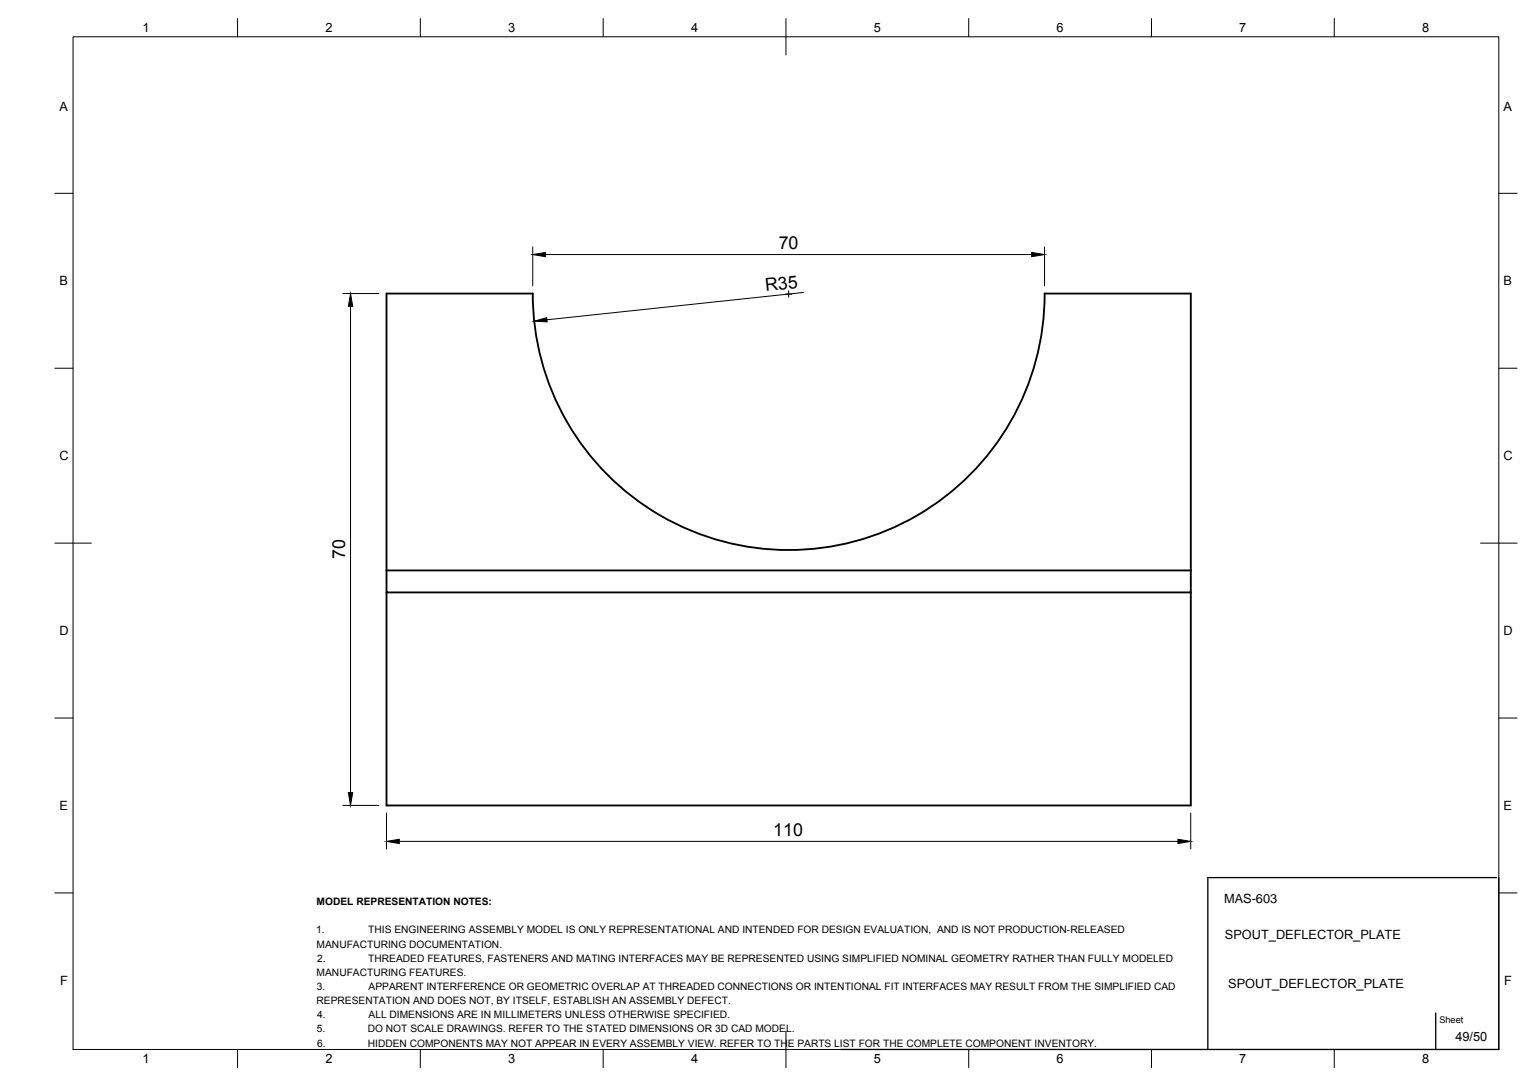
ISO-10303-21;
HEADER;
FILE_DESCRIPTION((''),'2;1');
FILE_NAME('SPOUT_DEFLECTOR_PLATE.step','2026-10-01T22:06:14-07:00',(''),(''),'','','');
FILE_SCHEMA (('AUTOMOTIVE_DESIGN { 1 0 10303 214 3 1 1 }'));
ENDSEC;
DATA;
#10=MECHANICAL_DESIGN_GEOMETRIC_PRESENTATION_REPRESENTATION('',(#1027,#1028),#50440);
#927=SHAPE_REPRESENTATION_RELATIONSHIP('SRR','None',#50661,#972) ;
#972=ADVANCED_BREP_SHAPE_REPRESENTATION('',(#1080,#1081),#50430) ;
#1027=STYLED_ITEM('',(#50889),#1080) ;
#1028=STYLED_ITEM('',(#50889),#1081) ;
#1080=MANIFOLD_SOLID_BREP('SPOUT_DEFLECTOR_PLATE',#28705) ;
#1081=MANIFOLD_SOLID_BREP('SPOUT_DEFLECTOR_PLATE',#28706) ;
#2276=PLANE('',#32170) ;
#2277=PLANE('',#32171) ;
#2278=PLANE('',#32172) ;
#2279=PLANE('',#32173) ;
#2280=PLANE('',#32174) ;
#2281=PLANE('',#32175) ;
#2282=PLANE('',#32176) ;
#2283=PLANE('',#32177) ;
#2284=PLANE('',#32178) ;
#2285=PLANE('',#32179) ;
#2286=PLANE('',#32180) ;
#2287=PLANE('',#32181) ;
#2288=PLANE('',#32182) ;
#3795=FACE_OUTER_BOUND('',#5635,.T.) ;
#3796=FACE_OUTER_BOUND('',#5636,.T.) ;
#3797=FACE_OUTER_BOUND('',#5637,.T.) ;
#3798=FACE_OUTER_BOUND('',#5638,.T.) ;
#3799=FACE_OUTER_BOUND('',#5639,.T.) ;
#3800=FACE_OUTER_BOUND('',#5640,.T.) ;
#3801=FACE_OUTER_BOUND('',#5641,.T.) ;
#3802=FACE_OUTER_BOUND('',#5642,.T.) ;
#3803=FACE_OUTER_BOUND('',#5643,.T.) ;
#3804=FACE_OUTER_BOUND('',#5644,.T.) ;
#3805=FACE_OUTER_BOUND('',#5645,.T.) ;
#3806=FACE_OUTER_BOUND('',#5646,.T.) ;
#3807=FACE_OUTER_BOUND('',#5647,.T.) ;
#3808=FACE_OUTER_BOUND('',#5648,.T.) ;
#5635=EDGE_LOOP('',(#26199,#26200,#26201,#26202)) ;
#5636=EDGE_LOOP('',(#26203,#26204,#26205,#26206,#26207,#26208)) ;
#5637=EDGE_LOOP('',(#26209,#26210,#26211,#26212)) ;
#5638=EDGE_LOOP('',(#26213,#26214,#26215,#26216)) ;
#5639=EDGE_LOOP('',(#26217,#26218,#26219,#26220)) ;
#5640=EDGE_LOOP('',(#26221,#26222,#26223,#26224)) ;
#5641=EDGE_LOOP('',(#26225,#26226,#26227,#26228)) ;
#5642=EDGE_LOOP('',(#26229,#26230,#26231,#26232,#26233,#26234)) ;
#5643=EDGE_LOOP('',(#26235,#26236,#26237,#26238)) ;
#5644=EDGE_LOOP('',(#26239,#26240,#26241,#26242)) ;
#5645=EDGE_LOOP('',(#26243,#26244,#26245,#26246)) ;
#5646=EDGE_LOOP('',(#26247,#26248,#26249,#26250)) ;
#5647=EDGE_LOOP('',(#26251,#26252,#26253,#26254)) ;
#5648=EDGE_LOOP('',(#26255,#26256,#26257,#26258)) ;
#8077=LINE('',#49780,#10549) ;
#8078=LINE('',#49784,#10550) ;
#8079=LINE('',#49788,#10551) ;
#8080=LINE('',#49790,#10552) ;
#8081=LINE('',#49792,#10553) ;
#8082=LINE('',#49794,#10554) ;
#8083=LINE('',#49795,#10555) ;
#8084=LINE('',#49798,#10556) ;
#8085=LINE('',#49799,#10557) ;
#8086=LINE('',#49802,#10558) ;
#8087=LINE('',#49803,#10559) ;
#8088=LINE('',#49807,#10560) ;
#8089=LINE('',#49808,#10561) ;
#8090=LINE('',#49809,#10562) ;
#8091=LINE('',#49811,#10563) ;
#8092=LINE('',#49813,#10564) ;
#8093=LINE('',#49818,#10565) ;
#8094=LINE('',#49820,#10566) ;
#8095=LINE('',#49822,#10567) ;
#8096=LINE('',#49823,#10568) ;
#8097=LINE('',#49827,#10569) ;
#8098=LINE('',#49829,#10570) ;
#8099=LINE('',#49831,#10571) ;
#8100=LINE('',#49832,#10572) ;
#8101=LINE('',#49834,#10573) ;
#8102=LINE('',#49835,#10574) ;
#8103=LINE('',#49837,#10575) ;
#8104=LINE('',#49839,#10576) ;
#10549=VECTOR('',#40638,1.) ;
#10550=VECTOR('',#40641,1.) ;
#10551=VECTOR('',#40646,1.) ;
#10552=VECTOR('',#40647,1.) ;
#10553=VECTOR('',#40648,1.) ;
#10554=VECTOR('',#40649,1.) ;
#10555=VECTOR('',#40650,1.) ;
#10556=VECTOR('',#40653,1.) ;
#10557=VECTOR('',#40654,1.) ;
#10558=VECTOR('',#40657,1.) ;
#10559=VECTOR('',#40658,1.) ;
#10560=VECTOR('',#40661,1.) ;
#10561=VECTOR('',#40662,1.) ;
#10562=VECTOR('',#40663,1.) ;
#10563=VECTOR('',#40666,1.) ;
#10564=VECTOR('',#40669,1.) ;
#10565=VECTOR('',#40674,1.) ;
#10566=VECTOR('',#40675,1.) ;
#10567=VECTOR('',#40676,1.) ;
#10568=VECTOR('',#40677,1.) ;
#10569=VECTOR('',#40680,1.) ;
#10570=VECTOR('',#40681,1.) ;
#10571=VECTOR('',#40682,1.) ;
#10572=VECTOR('',#40683,1.) ;
#10573=VECTOR('',#40686,1.) ;
#10574=VECTOR('',#40687,1.) ;
#10575=VECTOR('',#40690,1.) ;
#10576=VECTOR('',#40693,1.) ;
#11795=CIRCLE('',#32168,3.5) ;
#11796=CIRCLE('',#32169,3.5) ;
#14412=VERTEX_POINT('',#49778) ;
#14413=VERTEX_POINT('',#49779) ;
#14414=VERTEX_POINT('',#49781) ;
#14415=VERTEX_POINT('',#49783) ;
#14416=VERTEX_POINT('',#49787) ;
#14417=VERTEX_POINT('',#49789) ;
#14418=VERTEX_POINT('',#49791) ;
#14419=VERTEX_POINT('',#49793) ;
#14420=VERTEX_POINT('',#49797) ;
#14421=VERTEX_POINT('',#49801) ;
#14422=VERTEX_POINT('',#49805) ;
#14423=VERTEX_POINT('',#49806) ;
#14424=VERTEX_POINT('',#49816) ;
#14425=VERTEX_POINT('',#49817) ;
#14426=VERTEX_POINT('',#49819) ;
#14427=VERTEX_POINT('',#49821) ;
#14428=VERTEX_POINT('',#49825) ;
#14429=VERTEX_POINT('',#49826) ;
#14430=VERTEX_POINT('',#49828) ;
#14431=VERTEX_POINT('',#49830) ;
#18365=EDGE_CURVE('',#14412,#14413,#8077,.T.) ;
#18366=EDGE_CURVE('',#14414,#14412,#11795,.T.) ;
#18367=EDGE_CURVE('',#14415,#14414,#8078,.T.) ;
#18368=EDGE_CURVE('',#14413,#14415,#11796,.T.) ;
#18369=EDGE_CURVE('',#14416,#14412,#8079,.T.) ;
#18370=EDGE_CURVE('',#14416,#14417,#8080,.T.) ;
#18371=EDGE_CURVE('',#14418,#14417,#8081,.T.) ;
#18372=EDGE_CURVE('',#14419,#14418,#8082,.T.) ;
#18373=EDGE_CURVE('',#14414,#14419,#8083,.T.) ;
#18374=EDGE_CURVE('',#14413,#14420,#8084,.T.) ;
#18375=EDGE_CURVE('',#14420,#14416,#8085,.T.) ;
#18376=EDGE_CURVE('',#14419,#14421,#8086,.T.) ;
#18377=EDGE_CURVE('',#14421,#14415,#8087,.T.) ;
#18378=EDGE_CURVE('',#14422,#14423,#8088,.T.) ;
#18379=EDGE_CURVE('',#14423,#14418,#8089,.T.) ;
#18380=EDGE_CURVE('',#14417,#14422,#8090,.T.) ;
#18381=EDGE_CURVE('',#14421,#14423,#8091,.T.) ;
#18382=EDGE_CURVE('',#14420,#14422,#8092,.T.) ;
#18383=EDGE_CURVE('',#14424,#14425,#8093,.T.) ;
#18384=EDGE_CURVE('',#14425,#14426,#8094,.T.) ;
#18385=EDGE_CURVE('',#14426,#14427,#8095,.T.) ;
#18386=EDGE_CURVE('',#14427,#14424,#8096,.T.) ;
#18387=EDGE_CURVE('',#14428,#14429,#8097,.T.) ;
#18388=EDGE_CURVE('',#14429,#14430,#8098,.T.) ;
#18389=EDGE_CURVE('',#14430,#14431,#8099,.T.) ;
#18390=EDGE_CURVE('',#14431,#14428,#8100,.T.) ;
#18391=EDGE_CURVE('',#14427,#14430,#8101,.T.) ;
#18392=EDGE_CURVE('',#14424,#14429,#8102,.T.) ;
#18393=EDGE_CURVE('',#14426,#14431,#8103,.T.) ;
#18394=EDGE_CURVE('',#14425,#14428,#8104,.T.) ;
#26199=ORIENTED_EDGE('',*,*,#18365,.F.) ;
#26200=ORIENTED_EDGE('',*,*,#18366,.F.) ;
#26201=ORIENTED_EDGE('',*,*,#18367,.F.) ;
#26202=ORIENTED_EDGE('',*,*,#18368,.F.) ;
#26203=ORIENTED_EDGE('',*,*,#18366,.T.) ;
#26204=ORIENTED_EDGE('',*,*,#18369,.F.) ;
#26205=ORIENTED_EDGE('',*,*,#18370,.T.) ;
#26206=ORIENTED_EDGE('',*,*,#18371,.F.) ;
#26207=ORIENTED_EDGE('',*,*,#18372,.F.) ;
#26208=ORIENTED_EDGE('',*,*,#18373,.F.) ;
#26209=ORIENTED_EDGE('',*,*,#18365,.T.) ;
#26210=ORIENTED_EDGE('',*,*,#18374,.T.) ;
#26211=ORIENTED_EDGE('',*,*,#18375,.T.) ;
#26212=ORIENTED_EDGE('',*,*,#18369,.T.) ;
#26213=ORIENTED_EDGE('',*,*,#18367,.T.) ;
#26214=ORIENTED_EDGE('',*,*,#18373,.T.) ;
#26215=ORIENTED_EDGE('',*,*,#18376,.T.) ;
#26216=ORIENTED_EDGE('',*,*,#18377,.T.) ;
#26217=ORIENTED_EDGE('',*,*,#18378,.T.) ;
#26218=ORIENTED_EDGE('',*,*,#18379,.T.) ;
#26219=ORIENTED_EDGE('',*,*,#18371,.T.) ;
#26220=ORIENTED_EDGE('',*,*,#18380,.T.) ;
#26221=ORIENTED_EDGE('',*,*,#18372,.T.) ;
#26222=ORIENTED_EDGE('',*,*,#18379,.F.) ;
#26223=ORIENTED_EDGE('',*,*,#18381,.F.) ;
#26224=ORIENTED_EDGE('',*,*,#18376,.F.) ;
#26225=ORIENTED_EDGE('',*,*,#18382,.T.) ;
#26226=ORIENTED_EDGE('',*,*,#18380,.F.) ;
#26227=ORIENTED_EDGE('',*,*,#18370,.F.) ;
#26228=ORIENTED_EDGE('',*,*,#18375,.F.) ;
#26229=ORIENTED_EDGE('',*,*,#18368,.T.) ;
#26230=ORIENTED_EDGE('',*,*,#18377,.F.) ;
#26231=ORIENTED_EDGE('',*,*,#18381,.T.) ;
#26232=ORIENTED_EDGE('',*,*,#18378,.F.) ;
#26233=ORIENTED_EDGE('',*,*,#18382,.F.) ;
#26234=ORIENTED_EDGE('',*,*,#18374,.F.) ;
#26235=ORIENTED_EDGE('',*,*,#18383,.T.) ;
#26236=ORIENTED_EDGE('',*,*,#18384,.T.) ;
#26237=ORIENTED_EDGE('',*,*,#18385,.T.) ;
#26238=ORIENTED_EDGE('',*,*,#18386,.T.) ;
#26239=ORIENTED_EDGE('',*,*,#18387,.T.) ;
#26240=ORIENTED_EDGE('',*,*,#18388,.T.) ;
#26241=ORIENTED_EDGE('',*,*,#18389,.T.) ;
#26242=ORIENTED_EDGE('',*,*,#18390,.T.) ;
#26243=ORIENTED_EDGE('',*,*,#18391,.T.) ;
#26244=ORIENTED_EDGE('',*,*,#18388,.F.) ;
#26245=ORIENTED_EDGE('',*,*,#18392,.F.) ;
#26246=ORIENTED_EDGE('',*,*,#18386,.F.) ;
#26247=ORIENTED_EDGE('',*,*,#18393,.T.) ;
#26248=ORIENTED_EDGE('',*,*,#18389,.F.) ;
#26249=ORIENTED_EDGE('',*,*,#18391,.F.) ;
#26250=ORIENTED_EDGE('',*,*,#18385,.F.) ;
#26251=ORIENTED_EDGE('',*,*,#18394,.T.) ;
#26252=ORIENTED_EDGE('',*,*,#18390,.F.) ;
#26253=ORIENTED_EDGE('',*,*,#18393,.F.) ;
#26254=ORIENTED_EDGE('',*,*,#18384,.F.) ;
#26255=ORIENTED_EDGE('',*,*,#18392,.T.) ;
#26256=ORIENTED_EDGE('',*,*,#18387,.F.) ;
#26257=ORIENTED_EDGE('',*,*,#18394,.F.) ;
#26258=ORIENTED_EDGE('',*,*,#18383,.F.) ;
#27051=CYLINDRICAL_SURFACE('',#32167,3.5) ;
#28530=ADVANCED_FACE('',(#3795),#27051,.F.) ;
#28531=ADVANCED_FACE('',(#3796),#2276,.F.) ;
#28532=ADVANCED_FACE('',(#3797),#2277,.T.) ;
#28533=ADVANCED_FACE('',(#3798),#2278,.T.) ;
#28534=ADVANCED_FACE('',(#3799),#2279,.F.) ;
#28535=ADVANCED_FACE('',(#3800),#2280,.F.) ;
#28536=ADVANCED_FACE('',(#3801),#2281,.F.) ;
#28537=ADVANCED_FACE('',(#3802),#2282,.F.) ;
#28538=ADVANCED_FACE('',(#3803),#2283,.T.) ;
#28539=ADVANCED_FACE('',(#3804),#2284,.F.) ;
#28540=ADVANCED_FACE('',(#3805),#2285,.F.) ;
#28541=ADVANCED_FACE('',(#3806),#2286,.F.) ;
#28542=ADVANCED_FACE('',(#3807),#2287,.F.) ;
#28543=ADVANCED_FACE('',(#3808),#2288,.F.) ;
#28705=CLOSED_SHELL('',(#28530,#28531,#28532,#28533,#28534,#28535,#28536,
#28537)) ;
#28706=CLOSED_SHELL('',(#28538,#28539,#28540,#28541,#28542,#28543)) ;
#32166=AXIS2_PLACEMENT_3D('',#49776,#40634,#40635) ;
#32167=AXIS2_PLACEMENT_3D('',#49777,#40636,#40637) ;
#32168=AXIS2_PLACEMENT_3D('',#49782,#40639,#40640) ;
#32169=AXIS2_PLACEMENT_3D('',#49785,#40642,#40643) ;
#32170=AXIS2_PLACEMENT_3D('',#49786,#40644,#40645) ;
#32171=AXIS2_PLACEMENT_3D('',#49796,#40651,#40652) ;
#32172=AXIS2_PLACEMENT_3D('',#49800,#40655,#40656) ;
#32173=AXIS2_PLACEMENT_3D('',#49804,#40659,#40660) ;
#32174=AXIS2_PLACEMENT_3D('',#49810,#40664,#40665) ;
#32175=AXIS2_PLACEMENT_3D('',#49812,#40667,#40668) ;
#32176=AXIS2_PLACEMENT_3D('',#49814,#40670,#40671) ;
#32177=AXIS2_PLACEMENT_3D('',#49815,#40672,#40673) ;
#32178=AXIS2_PLACEMENT_3D('',#49824,#40678,#40679) ;
#32179=AXIS2_PLACEMENT_3D('',#49833,#40684,#40685) ;
#32180=AXIS2_PLACEMENT_3D('',#49836,#40688,#40689) ;
#32181=AXIS2_PLACEMENT_3D('',#49838,#40691,#40692) ;
#32182=AXIS2_PLACEMENT_3D('',#49840,#40694,#40695) ;
#40634=DIRECTION('axis',(0.,0.,1.)) ;
#40635=DIRECTION('refdir',(1.,0.,0.)) ;
#40636=DIRECTION('center_axis',(0.998052578482889,0.,-0.0623782861551805)) ;
#40637=DIRECTION('ref_axis',(-0.0623782861551805,1.22464679914735E-16,-0.998052578482889)) ;
#40638=DIRECTION('',(0.998052578482889,0.,-0.0623782861551805)) ;
#40639=DIRECTION('center_axis',(0.998052578482889,0.,-0.0623782861551805)) ;
#40640=DIRECTION('ref_axis',(0.0623782861551805,0.,0.998052578482889)) ;
#40641=DIRECTION('',(-0.998052578482889,0.,0.0623782861551805)) ;
#40642=DIRECTION('center_axis',(-0.998052578482889,0.,0.0623782861551805)) ;
#40643=DIRECTION('ref_axis',(0.0623782861551805,0.,0.998052578482889)) ;
#40644=DIRECTION('center_axis',(0.998052578482889,0.,-0.0623782861551805)) ;
#40645=DIRECTION('ref_axis',(-0.0623782861551805,0.,-0.998052578482889)) ;
#40646=DIRECTION('',(0.,-1.,0.)) ;
#40647=DIRECTION('',(-0.0623782861551805,0.,-0.998052578482889)) ;
#40648=DIRECTION('',(0.,1.,0.)) ;
#40649=DIRECTION('',(-0.0623782861551805,0.,-0.998052578482889)) ;
#40650=DIRECTION('',(0.,-1.,0.)) ;
#40651=DIRECTION('center_axis',(0.0623782861551805,0.,0.998052578482889)) ;
#40652=DIRECTION('ref_axis',(0.998052578482889,0.,-0.0623782861551805)) ;
#40653=DIRECTION('',(0.,1.,0.)) ;
#40654=DIRECTION('',(-0.998052578482889,0.,0.0623782861551805)) ;
#40655=DIRECTION('center_axis',(0.0623782861551805,0.,0.998052578482889)) ;
#40656=DIRECTION('ref_axis',(0.998052578482889,0.,-0.0623782861551805)) ;
#40657=DIRECTION('',(0.998052578482889,0.,-0.0623782861551805)) ;
#40658=DIRECTION('',(0.,1.,0.)) ;
#40659=DIRECTION('center_axis',(0.0623782861551805,0.,0.998052578482889)) ;
#40660=DIRECTION('ref_axis',(0.998052578482889,0.,-0.0623782861551805)) ;
#40661=DIRECTION('',(0.,-1.,0.)) ;
#40662=DIRECTION('',(-0.998052578482889,0.,0.0623782861551805)) ;
#40663=DIRECTION('',(0.998052578482889,0.,-0.0623782861551805)) ;
#40664=DIRECTION('center_axis',(0.,1.,0.)) ;
#40665=DIRECTION('ref_axis',(0.0623782861551805,0.,0.998052578482889)) ;
#40666=DIRECTION('',(-0.0623782861551805,0.,-0.998052578482889)) ;
#40667=DIRECTION('center_axis',(0.,-1.,0.)) ;
#40668=DIRECTION('ref_axis',(-0.0623782861551805,0.,-0.998052578482889)) ;
#40669=DIRECTION('',(-0.0623782861551805,0.,-0.998052578482889)) ;
#40670=DIRECTION('center_axis',(-0.998052578482889,0.,0.0623782861551805)) ;
#40671=DIRECTION('ref_axis',(0.0623782861551805,0.,0.998052578482889)) ;
#40672=DIRECTION('center_axis',(0.0623782861551805,0.,0.998052578482889)) ;
#40673=DIRECTION('ref_axis',(0.998052578482889,0.,-0.0623782861551805)) ;
#40674=DIRECTION('',(0.,1.,0.)) ;
#40675=DIRECTION('',(-0.998052578482889,0.,0.0623782861551805)) ;
#40676=DIRECTION('',(0.,-1.,0.)) ;
#40677=DIRECTION('',(0.998052578482889,0.,-0.0623782861551805)) ;
#40678=DIRECTION('center_axis',(0.0623782861551805,0.,0.998052578482889)) ;
#40679=DIRECTION('ref_axis',(0.998052578482889,0.,-0.0623782861551805)) ;
#40680=DIRECTION('',(0.,-1.,0.)) ;
#40681=DIRECTION('',(-0.998052578482889,0.,0.0623782861551805)) ;
#40682=DIRECTION('',(0.,1.,0.)) ;
#40683=DIRECTION('',(0.998052578482889,0.,-0.0623782861551805)) ;
#40684=DIRECTION('center_axis',(0.,1.,0.)) ;
#40685=DIRECTION('ref_axis',(0.0623782861551805,0.,0.998052578482889)) ;
#40686=DIRECTION('',(-0.0623782861551805,0.,-0.998052578482889)) ;
#40687=DIRECTION('',(-0.0623782861551805,0.,-0.998052578482889)) ;
#40688=DIRECTION('center_axis',(0.998052578482889,0.,-0.0623782861551805)) ;
#40689=DIRECTION('ref_axis',(-0.0623782861551805,0.,-0.998052578482889)) ;
#40690=DIRECTION('',(-0.0623782861551805,0.,-0.998052578482889)) ;
#40691=DIRECTION('center_axis',(0.,-1.,0.)) ;
#40692=DIRECTION('ref_axis',(-0.0623782861551805,0.,-0.998052578482889)) ;
#40693=DIRECTION('',(-0.0623782861551805,0.,-0.998052578482889)) ;
#40694=DIRECTION('center_axis',(-0.998052578482889,0.,0.0623782861551805)) ;
#40695=DIRECTION('ref_axis',(0.0623782861551805,0.,0.998052578482889)) ;
#49776=CARTESIAN_POINT('',(0.,0.,0.)) ;
#49777=CARTESIAN_POINT('Origin',(63.,0.,11.0625)) ;
#49778=CARTESIAN_POINT('',(64.2183240015431,3.49999336320522,10.9931840246901)) ;
#49779=CARTESIAN_POINT('',(64.6175450329363,3.49999336320522,10.968232710228)) ;
#49780=CARTESIAN_POINT('',(63.0004251688583,3.49999336320522,11.0693027017329)) ;
#49781=CARTESIAN_POINT('',(64.2183240015431,-3.49999336320522,10.9931840246901)) ;
#49782=CARTESIAN_POINT('Origin',(64.2178988326848,0.,10.9863813229572)) ;
#49783=CARTESIAN_POINT('',(64.6175450329363,-3.49999336320522,10.968232710228)) ;
#49784=CARTESIAN_POINT('',(63.0004251688583,-3.49999336320522,11.0693027017329)) ;
#49785=CARTESIAN_POINT('Origin',(64.617119864078,0.,10.9614300084951)) ;
#49786=CARTESIAN_POINT('Origin',(64.,0.,7.5)) ;
#49787=CARTESIAN_POINT('',(64.2183240015431,5.5,10.9931840246901)) ;
#49788=CARTESIAN_POINT('',(64.2183240015431,0.,10.9931840246901)) ;
#49789=CARTESIAN_POINT('',(63.7816759984569,5.5,4.00681597530989)) ;
#49790=CARTESIAN_POINT('',(64.,5.5,7.5)) ;
#49791=CARTESIAN_POINT('',(63.7816759984569,-5.5,4.00681597530989)) ;
#49792=CARTESIAN_POINT('',(63.7816759984569,0.,4.00681597530989)) ;
#49793=CARTESIAN_POINT('',(64.2183240015431,-5.5,10.9931840246901)) ;
#49794=CARTESIAN_POINT('',(64.,-5.5,7.5)) ;
#49795=CARTESIAN_POINT('',(64.2183240015431,0.,10.9931840246901)) ;
#49796=CARTESIAN_POINT('Origin',(64.4179345172397,0.,10.9807083674591)) ;
#49797=CARTESIAN_POINT('',(64.6175450329363,5.5,10.968232710228)) ;
#49798=CARTESIAN_POINT('',(64.6175450329363,0.,10.968232710228)) ;
#49799=CARTESIAN_POINT('',(64.4179345172397,5.5,10.9807083674591)) ;
#49800=CARTESIAN_POINT('Origin',(64.4179345172397,0.,10.9807083674591)) ;
#49801=CARTESIAN_POINT('',(64.6175450329363,-5.5,10.968232710228)) ;
#49802=CARTESIAN_POINT('',(64.4179345172397,-5.5,10.9807083674591)) ;
#49803=CARTESIAN_POINT('',(64.6175450329363,0.,10.968232710228)) ;
#49804=CARTESIAN_POINT('Origin',(63.9812865141534,0.,3.99434031807885)) ;
#49805=CARTESIAN_POINT('',(64.18089702985,5.5,3.98186466084782)) ;
#49806=CARTESIAN_POINT('',(64.18089702985,-5.5,3.98186466084782)) ;
#49807=CARTESIAN_POINT('',(64.18089702985,0.,3.98186466084782)) ;
#49808=CARTESIAN_POINT('',(63.9812865141534,-5.5,3.99434031807885)) ;
#49809=CARTESIAN_POINT('',(63.9812865141534,5.5,3.99434031807885)) ;
#49810=CARTESIAN_POINT('Origin',(64.1996105156966,-5.5,7.48752434276896)) ;
#49811=CARTESIAN_POINT('',(64.3992210313932,-5.5,7.47504868553793)) ;
#49812=CARTESIAN_POINT('Origin',(64.1996105156966,5.5,7.48752434276896)) ;
#49813=CARTESIAN_POINT('',(64.3992210313932,5.5,7.47504868553793)) ;
#49814=CARTESIAN_POINT('Origin',(64.3992210313932,0.,7.47504868553793)) ;
#49815=CARTESIAN_POINT('Origin',(67.5044881891305,0.,6.99376217138448)) ;
#49816=CARTESIAN_POINT('',(70.4986459245792,-5.5,6.80662731291894)) ;
#49817=CARTESIAN_POINT('',(70.4986459245792,5.5,6.80662731291894)) ;
#49818=CARTESIAN_POINT('',(70.4986459245792,0.,6.80662731291894)) ;
#49819=CARTESIAN_POINT('',(64.5103304536818,5.5,7.18089702985002)) ;
#49820=CARTESIAN_POINT('',(67.5044881891305,5.5,6.99376217138448)) ;
#49821=CARTESIAN_POINT('',(64.5103304536818,-5.5,7.18089702985002)) ;
#49822=CARTESIAN_POINT('',(64.5103304536818,0.,7.18089702985002)) ;
#49823=CARTESIAN_POINT('',(67.5044881891305,-5.5,6.99376217138448)) ;
#49824=CARTESIAN_POINT('Origin',(67.485774703284,0.,6.69434639783962)) ;
#49825=CARTESIAN_POINT('',(70.4799324387326,5.5,6.50721153937407)) ;
#49826=CARTESIAN_POINT('',(70.4799324387326,-5.5,6.50721153937407)) ;
#49827=CARTESIAN_POINT('',(70.4799324387326,0.,6.50721153937407)) ;
#49828=CARTESIAN_POINT('',(64.4916169678353,-5.5,6.88148125630516)) ;
#49829=CARTESIAN_POINT('',(67.485774703284,-5.5,6.69434639783962)) ;
#49830=CARTESIAN_POINT('',(64.4916169678353,5.5,6.88148125630516)) ;
#49831=CARTESIAN_POINT('',(64.4916169678353,0.,6.88148125630516)) ;
#49832=CARTESIAN_POINT('',(67.485774703284,5.5,6.69434639783962)) ;
#49833=CARTESIAN_POINT('Origin',(67.4951314462072,-5.5,6.84405428461205)) ;
#49834=CARTESIAN_POINT('',(64.5009737107586,-5.5,7.03118914307759)) ;
#49835=CARTESIAN_POINT('',(70.4892891816559,-5.5,6.65691942614651)) ;
#49836=CARTESIAN_POINT('Origin',(64.5009737107586,0.,7.03118914307759)) ;
#49837=CARTESIAN_POINT('',(64.5009737107586,5.5,7.03118914307759)) ;
#49838=CARTESIAN_POINT('Origin',(67.4951314462072,5.5,6.84405428461205)) ;
#49839=CARTESIAN_POINT('',(70.4892891816559,5.5,6.65691942614651)) ;
#49840=CARTESIAN_POINT('Origin',(70.4892891816559,0.,6.65691942614651)) ;
#50377=UNCERTAINTY_MEASURE_WITH_UNIT(LENGTH_MEASURE(0.001),#50441,
'DISTANCE_ACCURACY_VALUE',
'Maximum model space distance between geometric entities at asserted c
onnectivities') ;
#50387=UNCERTAINTY_MEASURE_WITH_UNIT(LENGTH_MEASURE(0.001),#50441,
'DISTANCE_ACCURACY_VALUE',
'Maximum model space distance between geometric entities at asserted c
onnectivities') ;
#50430=(
GEOMETRIC_REPRESENTATION_CONTEXT(3)
GLOBAL_UNCERTAINTY_ASSIGNED_CONTEXT((#50377))
GLOBAL_UNIT_ASSIGNED_CONTEXT((#50441,#50443,#50444))
REPRESENTATION_CONTEXT('','3D')
) ;
#50440=(
GEOMETRIC_REPRESENTATION_CONTEXT(3)
GLOBAL_UNCERTAINTY_ASSIGNED_CONTEXT((#50387))
GLOBAL_UNIT_ASSIGNED_CONTEXT((#50441,#50443,#50444))
REPRESENTATION_CONTEXT('','3D')
) ;
#50441=(
LENGTH_UNIT()
NAMED_UNIT(*)
SI_UNIT(.CENTI.,.METRE.)
) ;
#50443=(
NAMED_UNIT(*)
PLANE_ANGLE_UNIT()
SI_UNIT($,.RADIAN.)
) ;
#50444=(
NAMED_UNIT(*)
SI_UNIT($,.STERADIAN.)
SOLID_ANGLE_UNIT()
) ;
#50487=SHAPE_DEFINITION_REPRESENTATION(#50577,#50661) ;
#50577=PRODUCT_DEFINITION_SHAPE('',$,#50714) ;
#50661=SHAPE_REPRESENTATION('',(#32166),#50430) ;
#50671=PRODUCT_DEFINITION_CONTEXT('part definition',#50829,'design') ;
#50714=PRODUCT_DEFINITION('SPOUT_DEFLECTOR_PLATE',
'SPOUT_DEFLECTOR_PLATE',#50766,#50671) ;
#50766=PRODUCT_DEFINITION_FORMATION('',$,#50873) ;
#50829=APPLICATION_CONTEXT(
'Core Data for Automotive Mechanical Design Process') ;
#50830=PRODUCT_CONTEXT('part definition',#50829,'mechanical') ;
#50873=PRODUCT('SPOUT_DEFLECTOR_PLATE','SPOUT_DEFLECTOR_PLATE',$,(#50830)) ;
#50889=PRESENTATION_STYLE_ASSIGNMENT((#50896)) ;
#50896=SURFACE_STYLE_USAGE(.BOTH.,#50903) ;
#50903=SURFACE_SIDE_STYLE('',(#50910)) ;
#50910=SURFACE_STYLE_FILL_AREA(#50917) ;
#50917=FILL_AREA_STYLE('Stainless Steel - Satin',(#50924)) ;
#50924=FILL_AREA_STYLE_COLOUR('Stainless Steel - Satin',#50931) ;
#50931=COLOUR_RGB('Stainless Steel - Satin', 0.72549020, 0.75294118, 0.79215686) ;
ENDSEC;
END-ISO-10303-21;
